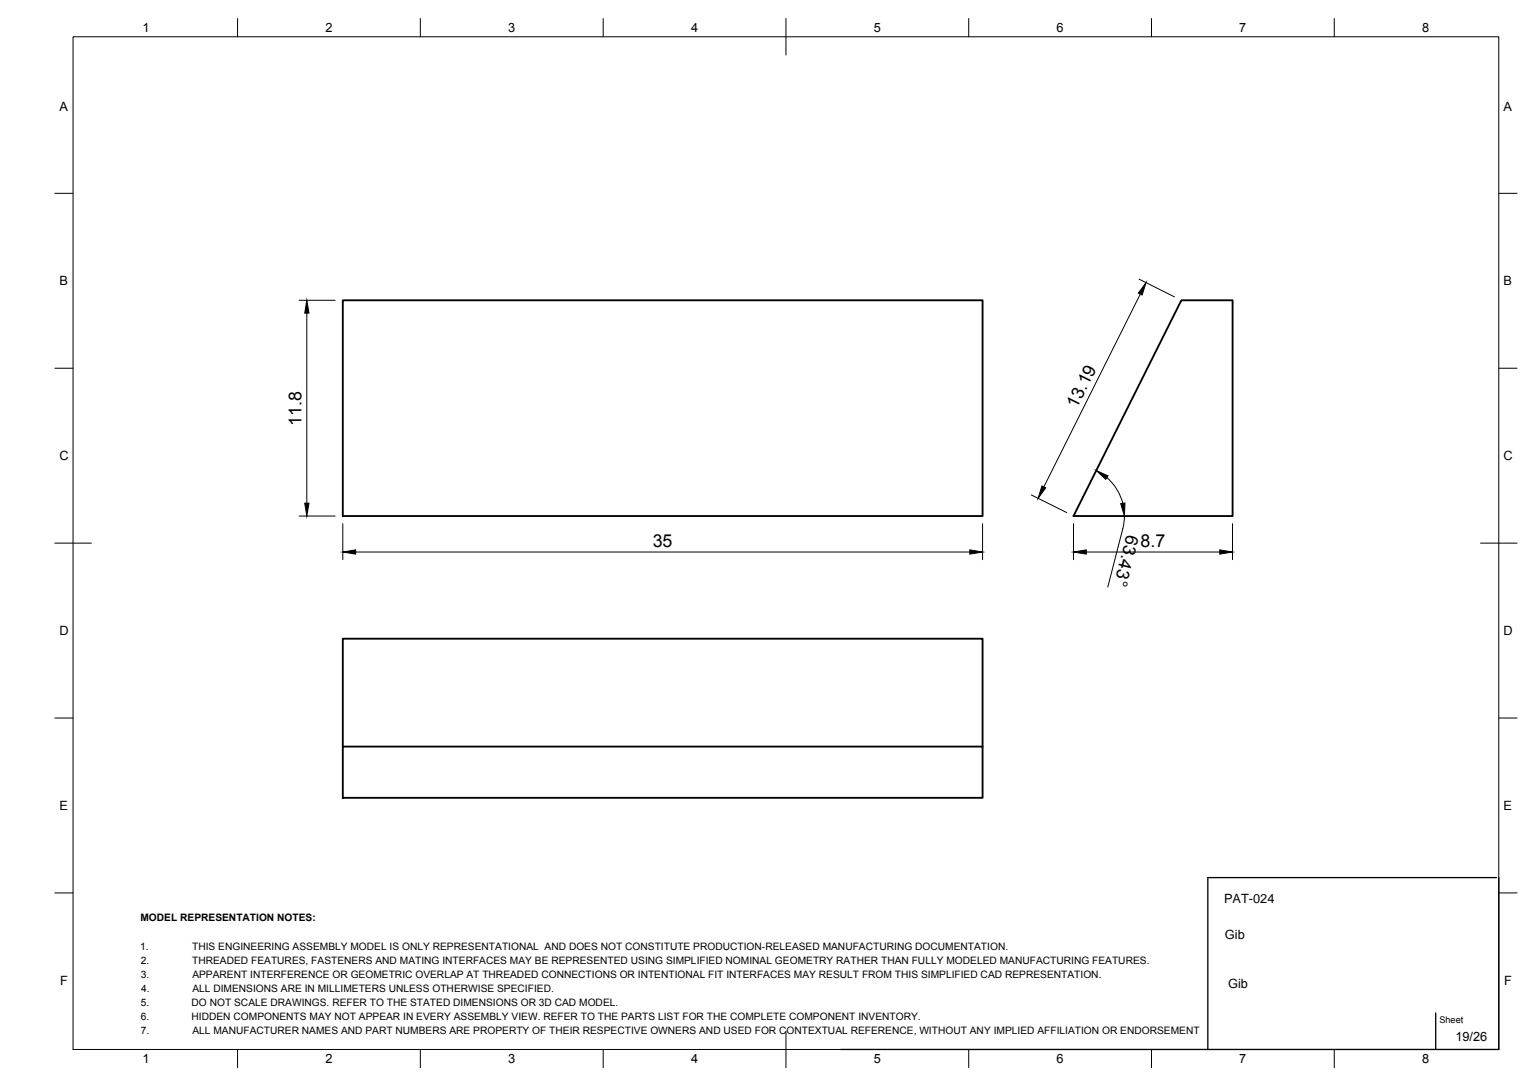
ISO-10303-21;
HEADER;
/* Generated by software containing ST-Developer
 * from STEP Tools, Inc. (www.steptools.com) 
 */

FILE_DESCRIPTION(
/* description */ ('Compact handwheel screw vise'),
/* implementation_level */ '2;1');

FILE_NAME(
/* name */ 'Gib.step',
/* time_stamp */ '2026-10-29T16:08:22-07:00',
/* author */ (''),
/* organization */ (''),
/* preprocessor_version */ 'ST-DEVELOPER v20.2',
/* originating_system */ 'Autodesk Translation Framework v15.17.0.0',
/* authorisation */ '');

FILE_SCHEMA (('AUTOMOTIVE_DESIGN { 1 0 10303 214 3 1 1 }'));
ENDSEC;

DATA;
#10=MECHANICAL_DESIGN_GEOMETRIC_PRESENTATION_REPRESENTATION('',(#665),#25074);
#601=SHAPE_REPRESENTATION_RELATIONSHIP('SRR','None',#25211,#629);
#629=ADVANCED_BREP_SHAPE_REPRESENTATION('',(#700),#25058);
#665=STYLED_ITEM('',(#25432),#700);
#700=MANIFOLD_SOLID_BREP('Body1',#8074);
#913=PLANE('',#8756);
#914=PLANE('',#8757);
#915=PLANE('',#8758);
#916=PLANE('',#8759);
#917=PLANE('',#8760);
#918=PLANE('',#8761);
#1183=FACE_OUTER_BOUND('',#1723,.T.);
#1184=FACE_OUTER_BOUND('',#1724,.T.);
#1185=FACE_OUTER_BOUND('',#1725,.T.);
#1186=FACE_OUTER_BOUND('',#1726,.T.);
#1187=FACE_OUTER_BOUND('',#1727,.T.);
#1188=FACE_OUTER_BOUND('',#1728,.T.);
#1723=EDGE_LOOP('',(#5851,#5852,#5853,#5854));
#1724=EDGE_LOOP('',(#5855,#5856,#5857,#5858));
#1725=EDGE_LOOP('',(#5859,#5860,#5861,#5862));
#1726=EDGE_LOOP('',(#5863,#5864,#5865,#5866));
#1727=EDGE_LOOP('',(#5867,#5868,#5869,#5870));
#1728=EDGE_LOOP('',(#5871,#5872,#5873,#5874));
#2229=LINE('',#12438,#2737);
#2230=LINE('',#12440,#2738);
#2231=LINE('',#12442,#2739);
#2232=LINE('',#12443,#2740);
#2233=LINE('',#12446,#2741);
#2234=LINE('',#12448,#2742);
#2235=LINE('',#12449,#2743);
#2236=LINE('',#12452,#2744);
#2237=LINE('',#12454,#2745);
#2238=LINE('',#12455,#2746);
#2239=LINE('',#12457,#2747);
#2240=LINE('',#12458,#2748);
#2737=VECTOR('',#10083,1.);
#2738=VECTOR('',#10084,1.);
#2739=VECTOR('',#10085,1.);
#2740=VECTOR('',#10086,1.);
#2741=VECTOR('',#10089,1.);
#2742=VECTOR('',#10090,1.);
#2743=VECTOR('',#10091,1.);
#2744=VECTOR('',#10094,1.);
#2745=VECTOR('',#10095,1.);
#2746=VECTOR('',#10096,1.);
#2747=VECTOR('',#10099,1.);
#2748=VECTOR('',#10100,1.);
#3572=VERTEX_POINT('',#12436);
#3573=VERTEX_POINT('',#12437);
#3574=VERTEX_POINT('',#12439);
#3575=VERTEX_POINT('',#12441);
#3576=VERTEX_POINT('',#12445);
#3577=VERTEX_POINT('',#12447);
#3578=VERTEX_POINT('',#12451);
#3579=VERTEX_POINT('',#12453);
#4412=EDGE_CURVE('',#3572,#3573,#2229,.T.);
#4413=EDGE_CURVE('',#3573,#3574,#2230,.T.);
#4414=EDGE_CURVE('',#3575,#3574,#2231,.T.);
#4415=EDGE_CURVE('',#3572,#3575,#2232,.T.);
#4416=EDGE_CURVE('',#3576,#3572,#2233,.T.);
#4417=EDGE_CURVE('',#3577,#3575,#2234,.T.);
#4418=EDGE_CURVE('',#3576,#3577,#2235,.T.);
#4419=EDGE_CURVE('',#3578,#3576,#2236,.T.);
#4420=EDGE_CURVE('',#3579,#3577,#2237,.T.);
#4421=EDGE_CURVE('',#3578,#3579,#2238,.T.);
#4422=EDGE_CURVE('',#3573,#3578,#2239,.T.);
#4423=EDGE_CURVE('',#3574,#3579,#2240,.T.);
#5851=ORIENTED_EDGE('',*,*,#4412,.T.);
#5852=ORIENTED_EDGE('',*,*,#4413,.T.);
#5853=ORIENTED_EDGE('',*,*,#4414,.F.);
#5854=ORIENTED_EDGE('',*,*,#4415,.F.);
#5855=ORIENTED_EDGE('',*,*,#4416,.T.);
#5856=ORIENTED_EDGE('',*,*,#4415,.T.);
#5857=ORIENTED_EDGE('',*,*,#4417,.F.);
#5858=ORIENTED_EDGE('',*,*,#4418,.F.);
#5859=ORIENTED_EDGE('',*,*,#4419,.T.);
#5860=ORIENTED_EDGE('',*,*,#4418,.T.);
#5861=ORIENTED_EDGE('',*,*,#4420,.F.);
#5862=ORIENTED_EDGE('',*,*,#4421,.F.);
#5863=ORIENTED_EDGE('',*,*,#4422,.T.);
#5864=ORIENTED_EDGE('',*,*,#4421,.T.);
#5865=ORIENTED_EDGE('',*,*,#4423,.F.);
#5866=ORIENTED_EDGE('',*,*,#4413,.F.);
#5867=ORIENTED_EDGE('',*,*,#4423,.T.);
#5868=ORIENTED_EDGE('',*,*,#4420,.T.);
#5869=ORIENTED_EDGE('',*,*,#4417,.T.);
#5870=ORIENTED_EDGE('',*,*,#4414,.T.);
#5871=ORIENTED_EDGE('',*,*,#4422,.F.);
#5872=ORIENTED_EDGE('',*,*,#4412,.F.);
#5873=ORIENTED_EDGE('',*,*,#4416,.F.);
#5874=ORIENTED_EDGE('',*,*,#4419,.F.);
#7753=ADVANCED_FACE('',(#1183),#913,.T.);
#7754=ADVANCED_FACE('',(#1184),#914,.T.);
#7755=ADVANCED_FACE('',(#1185),#915,.T.);
#7756=ADVANCED_FACE('',(#1186),#916,.T.);
#7757=ADVANCED_FACE('',(#1187),#917,.T.);
#7758=ADVANCED_FACE('',(#1188),#918,.F.);
#8074=CLOSED_SHELL('',(#7753,#7754,#7755,#7756,#7757,#7758));
#8755=AXIS2_PLACEMENT_3D('',#12434,#10079,#10080);
#8756=AXIS2_PLACEMENT_3D('',#12435,#10081,#10082);
#8757=AXIS2_PLACEMENT_3D('',#12444,#10087,#10088);
#8758=AXIS2_PLACEMENT_3D('',#12450,#10092,#10093);
#8759=AXIS2_PLACEMENT_3D('',#12456,#10097,#10098);
#8760=AXIS2_PLACEMENT_3D('',#12459,#10101,#10102);
#8761=AXIS2_PLACEMENT_3D('',#12460,#10103,#10104);
#10079=DIRECTION('axis',(0.,0.,1.));
#10080=DIRECTION('refdir',(1.,0.,0.));
#10081=DIRECTION('center_axis',(0.,0.,1.));
#10082=DIRECTION('ref_axis',(0.,-1.,0.));
#10083=DIRECTION('',(0.,-1.,0.));
#10084=DIRECTION('',(1.,0.,0.));
#10085=DIRECTION('',(0.,-1.,0.));
#10086=DIRECTION('',(1.,0.,0.));
#10087=DIRECTION('center_axis',(0.,1.,0.));
#10088=DIRECTION('ref_axis',(0.,0.,1.));
#10089=DIRECTION('',(0.,0.,1.));
#10090=DIRECTION('',(0.,0.,1.));
#10091=DIRECTION('',(1.,0.,0.));
#10092=DIRECTION('center_axis',(0.,0.,-1.));
#10093=DIRECTION('ref_axis',(0.,1.,0.));
#10094=DIRECTION('',(0.,1.,0.));
#10095=DIRECTION('',(0.,1.,0.));
#10096=DIRECTION('',(1.,0.,0.));
#10097=DIRECTION('center_axis',(0.,-0.894427190999916,0.447213595499958));
#10098=DIRECTION('ref_axis',(0.,-0.447213595499958,-0.894427190999916));
#10099=DIRECTION('',(0.,-0.447213595499958,-0.894427190999916));
#10100=DIRECTION('',(0.,-0.447213595499958,-0.894427190999916));
#10101=DIRECTION('center_axis',(1.,0.,0.));
#10102=DIRECTION('ref_axis',(0.,0.,-1.));
#10103=DIRECTION('center_axis',(1.,0.,0.));
#10104=DIRECTION('ref_axis',(0.,0.,-1.));
#12434=CARTESIAN_POINT('',(0.,0.,0.));
#12435=CARTESIAN_POINT('Origin',(11.,2.7,2.4));
#12436=CARTESIAN_POINT('',(11.,2.7,2.4));
#12437=CARTESIAN_POINT('',(11.,2.42,2.4));
#12438=CARTESIAN_POINT('',(11.,2.7,2.4));
#12439=CARTESIAN_POINT('',(14.5,2.42,2.4));
#12440=CARTESIAN_POINT('',(11.,2.42,2.4));
#12441=CARTESIAN_POINT('',(14.5,2.7,2.4));
#12442=CARTESIAN_POINT('',(14.5,2.7,2.4));
#12443=CARTESIAN_POINT('',(11.,2.7,2.4));
#12444=CARTESIAN_POINT('Origin',(11.,2.7,1.22));
#12445=CARTESIAN_POINT('',(11.,2.7,1.22));
#12446=CARTESIAN_POINT('',(11.,2.7,1.22));
#12447=CARTESIAN_POINT('',(14.5,2.7,1.22));
#12448=CARTESIAN_POINT('',(14.5,2.7,1.22));
#12449=CARTESIAN_POINT('',(11.,2.7,1.22));
#12450=CARTESIAN_POINT('Origin',(11.,1.83,1.22));
#12451=CARTESIAN_POINT('',(11.,1.83,1.22));
#12452=CARTESIAN_POINT('',(11.,1.83,1.22));
#12453=CARTESIAN_POINT('',(14.5,1.83,1.22));
#12454=CARTESIAN_POINT('',(14.5,1.83,1.22));
#12455=CARTESIAN_POINT('',(11.,1.83,1.22));
#12456=CARTESIAN_POINT('Origin',(11.,2.42,2.4));
#12457=CARTESIAN_POINT('',(11.,2.42,2.4));
#12458=CARTESIAN_POINT('',(14.5,2.42,2.4));
#12459=CARTESIAN_POINT('Origin',(14.5,2.265,1.81));
#12460=CARTESIAN_POINT('Origin',(11.,2.265,1.81));
#25024=UNCERTAINTY_MEASURE_WITH_UNIT(LENGTH_MEASURE(0.001),#25075,
'DISTANCE_ACCURACY_VALUE',
'Maximum model space distance between geometric entities at asserted c
onnectivities');
#25040=UNCERTAINTY_MEASURE_WITH_UNIT(LENGTH_MEASURE(0.001),#25075,
'DISTANCE_ACCURACY_VALUE',
'Maximum model space distance between geometric entities at asserted c
onnectivities');
#25058=(
GEOMETRIC_REPRESENTATION_CONTEXT(3)
GLOBAL_UNCERTAINTY_ASSIGNED_CONTEXT((#25024))
GLOBAL_UNIT_ASSIGNED_CONTEXT((#25075,#25077,#25078))
REPRESENTATION_CONTEXT('','3D')
);
#25074=(
GEOMETRIC_REPRESENTATION_CONTEXT(3)
GLOBAL_UNCERTAINTY_ASSIGNED_CONTEXT((#25040))
GLOBAL_UNIT_ASSIGNED_CONTEXT((#25075,#25077,#25078))
REPRESENTATION_CONTEXT('','3D')
);
#25075=(
LENGTH_UNIT()
NAMED_UNIT(*)
SI_UNIT(.CENTI.,.METRE.)
);
#25077=(
NAMED_UNIT(*)
PLANE_ANGLE_UNIT()
SI_UNIT($,.RADIAN.)
);
#25078=(
NAMED_UNIT(*)
SI_UNIT($,.STERADIAN.)
SOLID_ANGLE_UNIT()
);
#25096=SHAPE_DEFINITION_REPRESENTATION(#25134,#25211);
#25134=PRODUCT_DEFINITION_SHAPE('',$,#25245);
#25211=SHAPE_REPRESENTATION('',(#8755),#25058);
#25227=PRODUCT_DEFINITION_CONTEXT('part definition',#25328,'design');
#25245=PRODUCT_DEFINITION('Gib','Gib',#25278,#25227);
#25278=PRODUCT_DEFINITION_FORMATION('',$,#25347);
#25328=APPLICATION_CONTEXT(
'Core Data for Automotive Mechanical Design Process');
#25329=PRODUCT_CONTEXT('part definition',#25328,'mechanical');
#25347=PRODUCT('Gib','Gib','Gib',(#25329));
#25426=COLOUR_RGB('Sky Blue',0.24,0.69,0.87);
#25427=FILL_AREA_STYLE_COLOUR('',#25426);
#25428=FILL_AREA_STYLE('',(#25427));
#25429=SURFACE_STYLE_FILL_AREA(#25428);
#25430=SURFACE_SIDE_STYLE('',(#25429));
#25431=SURFACE_STYLE_USAGE(.BOTH.,#25430);
#25432=PRESENTATION_STYLE_ASSIGNMENT((#25431));
ENDSEC;
END-ISO-10303-21;
